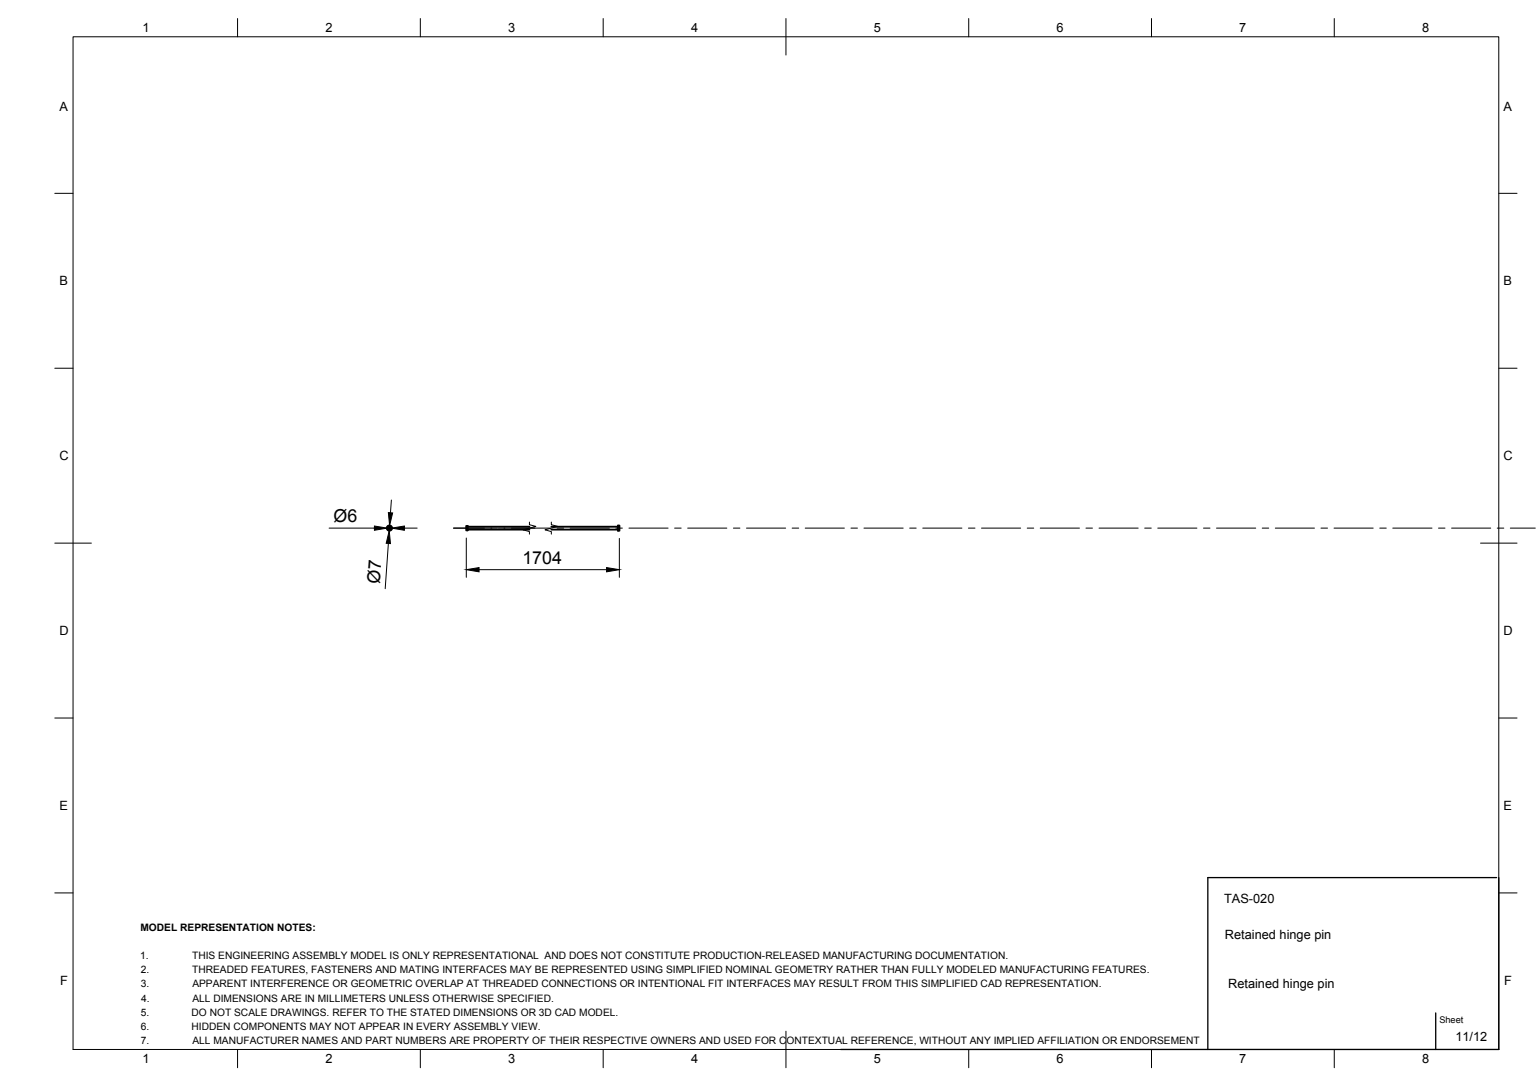
ISO-10303-21;
HEADER;
/* Generated by software containing ST-Developer
 * from STEP Tools, Inc. (www.steptools.com) 
 */

FILE_DESCRIPTION(
/* description */ (''),
/* implementation_level */ '2;1');

FILE_NAME(
/* name */ 'Retained hinge pin.step',
/* time_stamp */ '2026-11-15T17:46:57-08:00',
/* author */ (''),
/* organization */ (''),
/* preprocessor_version */ 'ST-DEVELOPER v20.2',
/* originating_system */ 'Autodesk Translation Framework v15.17.0.0',
/* authorisation */ '');

FILE_SCHEMA (('AUTOMOTIVE_DESIGN { 1 0 10303 214 3 1 1 }'));
ENDSEC;

DATA;
#10=MECHANICAL_DESIGN_GEOMETRIC_PRESENTATION_REPRESENTATION('',(#383),#12963);
#359=SHAPE_REPRESENTATION_RELATIONSHIP('SRR','None',#13043,#371);
#371=ADVANCED_BREP_SHAPE_REPRESENTATION('',(#395),#12959);
#383=STYLED_ITEM('',(#13112),#395);
#395=MANIFOLD_SOLID_BREP('Body1',#4817);
#435=FACE_BOUND('',#1003,.T.);
#436=FACE_BOUND('',#1006,.T.);
#548=PLANE('',#5164);
#549=PLANE('',#5169);
#550=PLANE('',#5174);
#551=PLANE('',#5176);
#710=FACE_OUTER_BOUND('',#1002,.T.);
#711=FACE_OUTER_BOUND('',#1004,.T.);
#712=FACE_OUTER_BOUND('',#1005,.T.);
#713=FACE_OUTER_BOUND('',#1007,.T.);
#714=FACE_OUTER_BOUND('',#1008,.T.);
#715=FACE_OUTER_BOUND('',#1009,.T.);
#716=FACE_OUTER_BOUND('',#1010,.T.);
#1002=EDGE_LOOP('',(#3796));
#1003=EDGE_LOOP('',(#3797));
#1004=EDGE_LOOP('',(#3798,#3799,#3800,#3801));
#1005=EDGE_LOOP('',(#3802));
#1006=EDGE_LOOP('',(#3803));
#1007=EDGE_LOOP('',(#3804,#3805,#3806,#3807));
#1008=EDGE_LOOP('',(#3808));
#1009=EDGE_LOOP('',(#3809,#3810,#3811,#3812));
#1010=EDGE_LOOP('',(#3813));
#1406=LINE('',#7243,#1808);
#1407=LINE('',#7251,#1809);
#1408=LINE('',#7255,#1810);
#1808=VECTOR('',#6051,0.3);
#1809=VECTOR('',#6060,0.35);
#1810=VECTOR('',#6067,0.2);
#1992=CIRCLE('',#5165,0.3);
#1993=CIRCLE('',#5166,0.2);
#1994=CIRCLE('',#5168,0.3);
#1995=CIRCLE('',#5170,0.35);
#1996=CIRCLE('',#5171,0.2);
#1997=CIRCLE('',#5173,0.35);
#2240=VERTEX_POINT('',#7236);
#2241=VERTEX_POINT('',#7238);
#2242=VERTEX_POINT('',#7241);
#2243=VERTEX_POINT('',#7245);
#2244=VERTEX_POINT('',#7247);
#2245=VERTEX_POINT('',#7250);
#2794=EDGE_CURVE('',#2240,#2240,#1992,.T.);
#2795=EDGE_CURVE('',#2241,#2241,#1993,.T.);
#2796=EDGE_CURVE('',#2242,#2242,#1994,.T.);
#2797=EDGE_CURVE('',#2242,#2240,#1406,.T.);
#2798=EDGE_CURVE('',#2243,#2243,#1995,.T.);
#2799=EDGE_CURVE('',#2244,#2244,#1996,.T.);
#2800=EDGE_CURVE('',#2243,#2245,#1407,.T.);
#2801=EDGE_CURVE('',#2245,#2245,#1997,.T.);
#2802=EDGE_CURVE('',#2241,#2244,#1408,.T.);
#3796=ORIENTED_EDGE('',*,*,#2794,.F.);
#3797=ORIENTED_EDGE('',*,*,#2795,.F.);
#3798=ORIENTED_EDGE('',*,*,#2796,.F.);
#3799=ORIENTED_EDGE('',*,*,#2797,.T.);
#3800=ORIENTED_EDGE('',*,*,#2794,.T.);
#3801=ORIENTED_EDGE('',*,*,#2797,.F.);
#3802=ORIENTED_EDGE('',*,*,#2798,.T.);
#3803=ORIENTED_EDGE('',*,*,#2799,.F.);
#3804=ORIENTED_EDGE('',*,*,#2798,.F.);
#3805=ORIENTED_EDGE('',*,*,#2800,.T.);
#3806=ORIENTED_EDGE('',*,*,#2801,.T.);
#3807=ORIENTED_EDGE('',*,*,#2800,.F.);
#3808=ORIENTED_EDGE('',*,*,#2801,.F.);
#3809=ORIENTED_EDGE('',*,*,#2795,.T.);
#3810=ORIENTED_EDGE('',*,*,#2802,.T.);
#3811=ORIENTED_EDGE('',*,*,#2799,.T.);
#3812=ORIENTED_EDGE('',*,*,#2802,.F.);
#3813=ORIENTED_EDGE('',*,*,#2796,.T.);
#4463=CYLINDRICAL_SURFACE('',#5167,0.3);
#4464=CYLINDRICAL_SURFACE('',#5172,0.35);
#4465=CYLINDRICAL_SURFACE('',#5175,0.2);
#4691=ADVANCED_FACE('',(#710,#435),#548,.F.);
#4692=ADVANCED_FACE('',(#711),#4463,.T.);
#4693=ADVANCED_FACE('',(#712,#436),#549,.T.);
#4694=ADVANCED_FACE('',(#713),#4464,.T.);
#4695=ADVANCED_FACE('',(#714),#550,.F.);
#4696=ADVANCED_FACE('',(#715),#4465,.T.);
#4697=ADVANCED_FACE('',(#716),#551,.T.);
#4817=CLOSED_SHELL('',(#4691,#4692,#4693,#4694,#4695,#4696,#4697));
#5163=AXIS2_PLACEMENT_3D('',#7234,#6039,#6040);
#5164=AXIS2_PLACEMENT_3D('',#7235,#6041,#6042);
#5165=AXIS2_PLACEMENT_3D('',#7237,#6043,#6044);
#5166=AXIS2_PLACEMENT_3D('',#7239,#6045,#6046);
#5167=AXIS2_PLACEMENT_3D('',#7240,#6047,#6048);
#5168=AXIS2_PLACEMENT_3D('',#7242,#6049,#6050);
#5169=AXIS2_PLACEMENT_3D('',#7244,#6052,#6053);
#5170=AXIS2_PLACEMENT_3D('',#7246,#6054,#6055);
#5171=AXIS2_PLACEMENT_3D('',#7248,#6056,#6057);
#5172=AXIS2_PLACEMENT_3D('',#7249,#6058,#6059);
#5173=AXIS2_PLACEMENT_3D('',#7252,#6061,#6062);
#5174=AXIS2_PLACEMENT_3D('',#7253,#6063,#6064);
#5175=AXIS2_PLACEMENT_3D('',#7254,#6065,#6066);
#5176=AXIS2_PLACEMENT_3D('',#7256,#6068,#6069);
#6039=DIRECTION('axis',(0.,0.,1.));
#6040=DIRECTION('refdir',(1.,0.,0.));
#6041=DIRECTION('center_axis',(0.,0.,1.));
#6042=DIRECTION('ref_axis',(1.,0.,0.));
#6043=DIRECTION('center_axis',(0.,0.,1.));
#6044=DIRECTION('ref_axis',(1.,0.,0.));
#6045=DIRECTION('center_axis',(0.,0.,-1.));
#6046=DIRECTION('ref_axis',(1.,0.,0.));
#6047=DIRECTION('center_axis',(0.,0.,1.));
#6048=DIRECTION('ref_axis',(1.,0.,0.));
#6049=DIRECTION('center_axis',(0.,0.,1.));
#6050=DIRECTION('ref_axis',(1.,0.,0.));
#6051=DIRECTION('',(0.,0.,-1.));
#6052=DIRECTION('center_axis',(0.,0.,1.));
#6053=DIRECTION('ref_axis',(1.,0.,0.));
#6054=DIRECTION('center_axis',(0.,0.,1.));
#6055=DIRECTION('ref_axis',(1.,0.,0.));
#6056=DIRECTION('center_axis',(0.,0.,1.));
#6057=DIRECTION('ref_axis',(1.,0.,0.));
#6058=DIRECTION('center_axis',(0.,0.,1.));
#6059=DIRECTION('ref_axis',(1.,0.,0.));
#6060=DIRECTION('',(0.,0.,-1.));
#6061=DIRECTION('center_axis',(0.,0.,1.));
#6062=DIRECTION('ref_axis',(1.,0.,0.));
#6063=DIRECTION('center_axis',(0.,0.,1.));
#6064=DIRECTION('ref_axis',(1.,0.,0.));
#6065=DIRECTION('center_axis',(0.,0.,1.));
#6066=DIRECTION('ref_axis',(1.,0.,0.));
#6067=DIRECTION('',(0.,0.,-1.));
#6068=DIRECTION('center_axis',(0.,0.,1.));
#6069=DIRECTION('ref_axis',(1.,0.,0.));
#7234=CARTESIAN_POINT('',(0.,0.,0.));
#7235=CARTESIAN_POINT('Origin',(0.,0.,170.));
#7236=CARTESIAN_POINT('',(-0.3,-3.67394039744206E-17,170.));
#7237=CARTESIAN_POINT('Origin',(0.,0.,170.));
#7238=CARTESIAN_POINT('',(-0.2,2.44929359829471E-17,170.));
#7239=CARTESIAN_POINT('Origin',(0.,0.,170.));
#7240=CARTESIAN_POINT('Origin',(0.,0.,170.));
#7241=CARTESIAN_POINT('',(-0.3,-3.67394039744206E-17,170.2));
#7242=CARTESIAN_POINT('Origin',(0.,0.,170.2));
#7243=CARTESIAN_POINT('',(-0.3,-3.67394039744206E-17,170.));
#7244=CARTESIAN_POINT('Origin',(0.,0.,0.));
#7245=CARTESIAN_POINT('',(-0.35,-4.28626379701574E-17,0.));
#7246=CARTESIAN_POINT('Origin',(0.,0.,0.));
#7247=CARTESIAN_POINT('',(-0.2,-2.44929359829471E-17,0.));
#7248=CARTESIAN_POINT('Origin',(0.,0.,0.));
#7249=CARTESIAN_POINT('Origin',(0.,0.,-0.2));
#7250=CARTESIAN_POINT('',(-0.35,-4.28626379701574E-17,-0.2));
#7251=CARTESIAN_POINT('',(-0.35,-4.28626379701574E-17,-0.2));
#7252=CARTESIAN_POINT('Origin',(0.,0.,-0.2));
#7253=CARTESIAN_POINT('Origin',(0.,0.,-0.2));
#7254=CARTESIAN_POINT('Origin',(0.,0.,0.));
#7255=CARTESIAN_POINT('',(-0.2,-2.44929359829471E-17,0.));
#7256=CARTESIAN_POINT('Origin',(0.,0.,170.2));
#12945=UNCERTAINTY_MEASURE_WITH_UNIT(LENGTH_MEASURE(0.001),#12964,
'DISTANCE_ACCURACY_VALUE',
'Maximum model space distance between geometric entities at asserted c
onnectivities');
#12949=UNCERTAINTY_MEASURE_WITH_UNIT(LENGTH_MEASURE(0.001),#12964,
'DISTANCE_ACCURACY_VALUE',
'Maximum model space distance between geometric entities at asserted c
onnectivities');
#12959=(
GEOMETRIC_REPRESENTATION_CONTEXT(3)
GLOBAL_UNCERTAINTY_ASSIGNED_CONTEXT((#12945))
GLOBAL_UNIT_ASSIGNED_CONTEXT((#12964,#12966,#12967))
REPRESENTATION_CONTEXT('','3D')
);
#12963=(
GEOMETRIC_REPRESENTATION_CONTEXT(3)
GLOBAL_UNCERTAINTY_ASSIGNED_CONTEXT((#12949))
GLOBAL_UNIT_ASSIGNED_CONTEXT((#12964,#12966,#12967))
REPRESENTATION_CONTEXT('','3D')
);
#12964=(
LENGTH_UNIT()
NAMED_UNIT(*)
SI_UNIT(.CENTI.,.METRE.)
);
#12966=(
NAMED_UNIT(*)
PLANE_ANGLE_UNIT()
SI_UNIT($,.RADIAN.)
);
#12967=(
NAMED_UNIT(*)
SI_UNIT($,.STERADIAN.)
SOLID_ANGLE_UNIT()
);
#12977=SHAPE_DEFINITION_REPRESENTATION(#12990,#13043);
#12990=PRODUCT_DEFINITION_SHAPE('',$,#13057);
#13043=SHAPE_REPRESENTATION('',(#5163),#12959);
#13047=PRODUCT_DEFINITION_CONTEXT('part definition',#13088,'design');
#13057=PRODUCT_DEFINITION('Retained hinge pin','Retained hinge pin',#13070,
#13047);
#13070=PRODUCT_DEFINITION_FORMATION('',$,#13099);
#13088=APPLICATION_CONTEXT(
'Core Data for Automotive Mechanical Design Process');
#13089=PRODUCT_CONTEXT('part definition',#13088,'mechanical');
#13099=PRODUCT('Retained hinge pin','Retained hinge pin',$,(#13089));
#13112=PRESENTATION_STYLE_ASSIGNMENT((#13125));
#13125=SURFACE_STYLE_USAGE(.BOTH.,#13138);
#13138=SURFACE_SIDE_STYLE('',(#13151));
#13151=SURFACE_STYLE_FILL_AREA(#13164);
#13164=FILL_AREA_STYLE('Retained hinge pin finish',(#13177));
#13177=FILL_AREA_STYLE_COLOUR('Retained hinge pin finish',#13190);
#13190=COLOUR_RGB('Retained hinge pin finish',0.294117647058824,0.317647058823529,
0.36078431372549);
ENDSEC;
END-ISO-10303-21;
